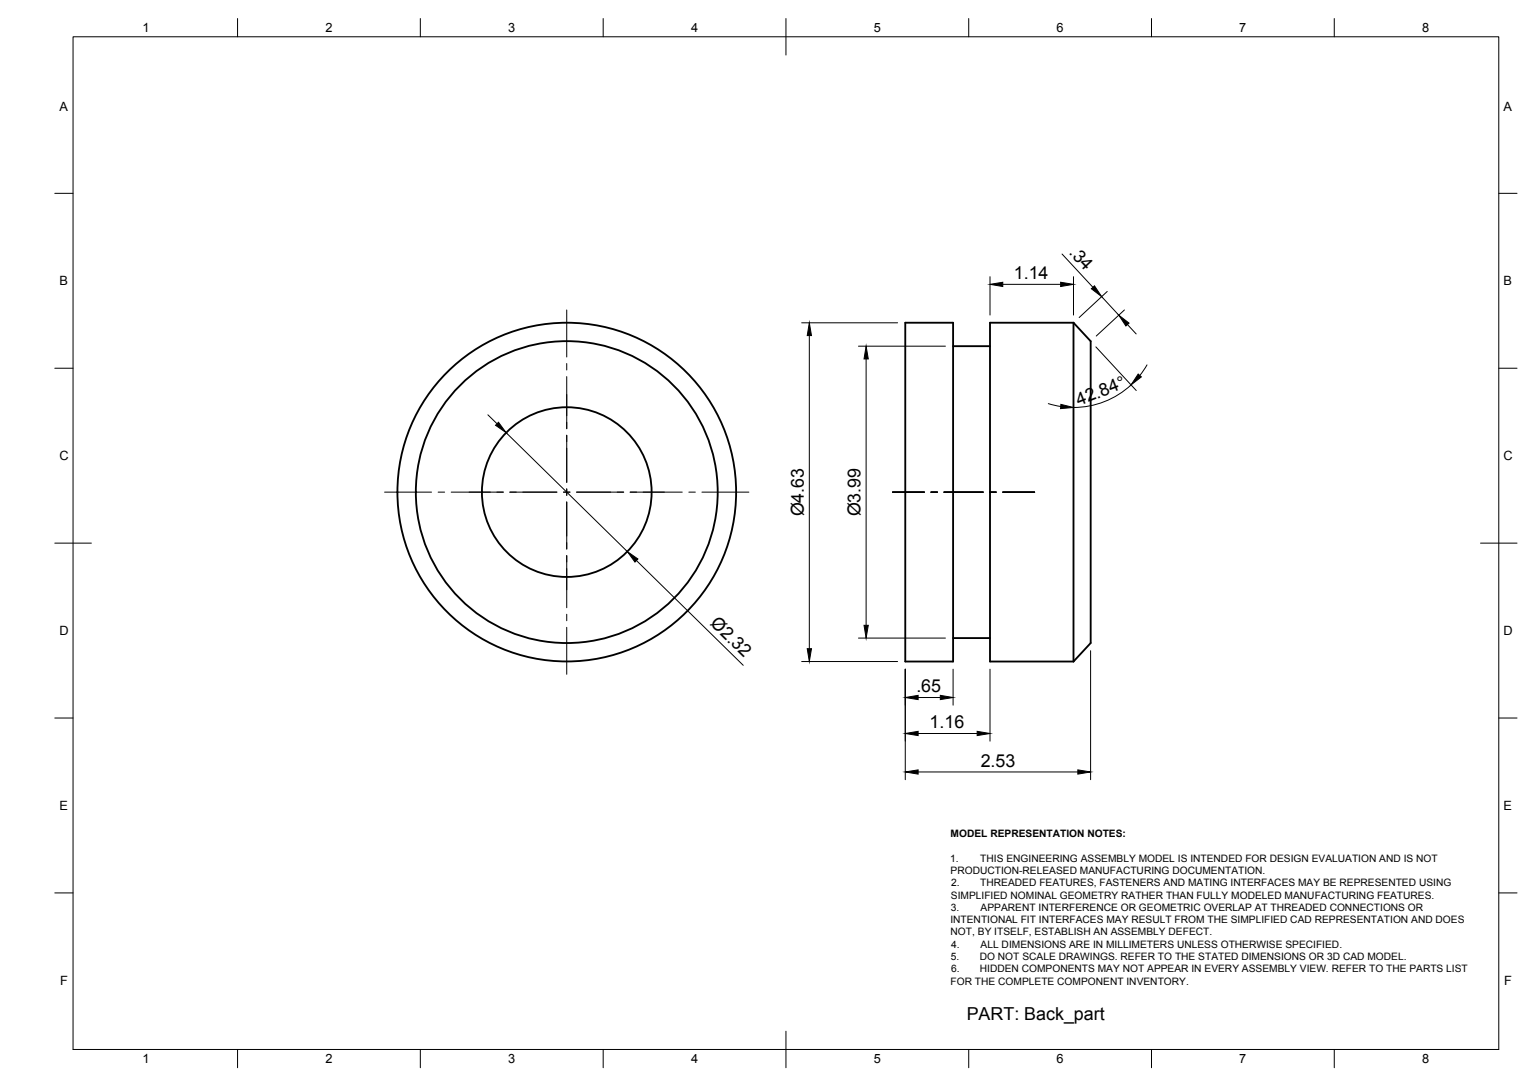
ISO-10303-21;
HEADER;
/* Generated by software containing ST-Developer
 * from STEP Tools, Inc. (www.steptools.com) 
 */

FILE_DESCRIPTION(
/* description */ (''),
/* implementation_level */ '2;1');

FILE_NAME(
/* name */ 'Back_part.step',
/* time_stamp */ '2026-10-05T00:51:14-07:00',
/* author */ (''),
/* organization */ (''),
/* preprocessor_version */ 'ST-DEVELOPER v20.2',
/* originating_system */ 'Autodesk Translation Framework v15.15.0.0',
/* authorisation */ '');

FILE_SCHEMA (('AUTOMOTIVE_DESIGN { 1 0 10303 214 3 1 1 }'));
ENDSEC;

DATA;
#10=MECHANICAL_DESIGN_GEOMETRIC_PRESENTATION_REPRESENTATION('',(#391),#4613);
#58=CONICAL_SURFACE('',#1792,2.1899902410121,0.823106104053138);
#59=CONICAL_SURFACE('',#1807,1.54725736664436,1.55720056407458);
#80=FACE_BOUND('',#574,.T.);
#81=FACE_BOUND('',#577,.T.);
#82=FACE_BOUND('',#580,.T.);
#83=FACE_BOUND('',#584,.T.);
#110=PLANE('',#1797);
#111=PLANE('',#1801);
#112=PLANE('',#1805);
#113=PLANE('',#1811);
#199=LINE('',#2684,#282);
#200=LINE('',#2689,#283);
#201=LINE('',#2696,#284);
#202=LINE('',#2703,#285);
#203=LINE('',#2710,#286);
#204=LINE('',#2714,#287);
#282=VECTOR('',#2142,2.1899902410121);
#283=VECTOR('',#2149,2.3164003912567);
#284=VECTOR('',#2158,1.99619194538056);
#285=VECTOR('',#2167,2.3164003912567);
#286=VECTOR('',#2176,1.54725736664436);
#287=VECTOR('',#2181,1.16083957311848);
#350=CYLINDRICAL_SURFACE('',#1795,2.3164003912567);
#351=CYLINDRICAL_SURFACE('',#1799,1.99619194538056);
#352=CYLINDRICAL_SURFACE('',#1803,2.3164003912567);
#353=CYLINDRICAL_SURFACE('',#1809,1.16083957311848);
#375=SHAPE_REPRESENTATION_RELATIONSHIP('SRR','None',#4649,#383);
#383=ADVANCED_BREP_SHAPE_REPRESENTATION('',(#399),#4609);
#391=STYLED_ITEM('',(#4695),#399);
#399=MANIFOLD_SOLID_BREP('Body1',#1598);
#452=FACE_OUTER_BOUND('',#571,.T.);
#453=FACE_OUTER_BOUND('',#572,.T.);
#454=FACE_OUTER_BOUND('',#573,.T.);
#455=FACE_OUTER_BOUND('',#575,.T.);
#456=FACE_OUTER_BOUND('',#576,.T.);
#457=FACE_OUTER_BOUND('',#578,.T.);
#458=FACE_OUTER_BOUND('',#579,.T.);
#459=FACE_OUTER_BOUND('',#581,.T.);
#460=FACE_OUTER_BOUND('',#582,.T.);
#461=FACE_OUTER_BOUND('',#583,.T.);
#571=EDGE_LOOP('',(#1245,#1246,#1247,#1248));
#572=EDGE_LOOP('',(#1249,#1250,#1251,#1252));
#573=EDGE_LOOP('',(#1253));
#574=EDGE_LOOP('',(#1254));
#575=EDGE_LOOP('',(#1255,#1256,#1257,#1258));
#576=EDGE_LOOP('',(#1259));
#577=EDGE_LOOP('',(#1260));
#578=EDGE_LOOP('',(#1261,#1262,#1263,#1264));
#579=EDGE_LOOP('',(#1265));
#580=EDGE_LOOP('',(#1266));
#581=EDGE_LOOP('',(#1267,#1268,#1269,#1270));
#582=EDGE_LOOP('',(#1271,#1272,#1273,#1274));
#583=EDGE_LOOP('',(#1275));
#584=EDGE_LOOP('',(#1276));
#685=CIRCLE('',#1793,2.3164003912567);
#686=CIRCLE('',#1794,2.06358009076751);
#687=CIRCLE('',#1796,2.3164003912567);
#688=CIRCLE('',#1798,1.99619194538056);
#689=CIRCLE('',#1800,1.99619194538056);
#690=CIRCLE('',#1802,2.3164003912567);
#691=CIRCLE('',#1804,2.3164003912567);
#692=CIRCLE('',#1806,1.93367516017024);
#693=CIRCLE('',#1808,1.16083957311848);
#694=CIRCLE('',#1810,1.16083957311848);
#786=VERTEX_POINT('',#2681);
#787=VERTEX_POINT('',#2683);
#788=VERTEX_POINT('',#2687);
#789=VERTEX_POINT('',#2691);
#790=VERTEX_POINT('',#2694);
#791=VERTEX_POINT('',#2698);
#792=VERTEX_POINT('',#2701);
#793=VERTEX_POINT('',#2705);
#794=VERTEX_POINT('',#2708);
#795=VERTEX_POINT('',#2712);
#950=EDGE_CURVE('',#786,#786,#685,.T.);
#951=EDGE_CURVE('',#786,#787,#199,.T.);
#952=EDGE_CURVE('',#787,#787,#686,.T.);
#953=EDGE_CURVE('',#788,#788,#687,.T.);
#954=EDGE_CURVE('',#788,#786,#200,.T.);
#955=EDGE_CURVE('',#789,#789,#688,.T.);
#956=EDGE_CURVE('',#790,#790,#689,.T.);
#957=EDGE_CURVE('',#790,#789,#201,.T.);
#958=EDGE_CURVE('',#791,#791,#690,.T.);
#959=EDGE_CURVE('',#792,#792,#691,.T.);
#960=EDGE_CURVE('',#792,#791,#202,.T.);
#961=EDGE_CURVE('',#793,#793,#692,.T.);
#962=EDGE_CURVE('',#794,#794,#693,.T.);
#963=EDGE_CURVE('',#794,#793,#203,.T.);
#964=EDGE_CURVE('',#795,#795,#694,.T.);
#965=EDGE_CURVE('',#795,#794,#204,.T.);
#1245=ORIENTED_EDGE('',*,*,#950,.F.);
#1246=ORIENTED_EDGE('',*,*,#951,.T.);
#1247=ORIENTED_EDGE('',*,*,#952,.T.);
#1248=ORIENTED_EDGE('',*,*,#951,.F.);
#1249=ORIENTED_EDGE('',*,*,#953,.F.);
#1250=ORIENTED_EDGE('',*,*,#954,.T.);
#1251=ORIENTED_EDGE('',*,*,#950,.T.);
#1252=ORIENTED_EDGE('',*,*,#954,.F.);
#1253=ORIENTED_EDGE('',*,*,#953,.T.);
#1254=ORIENTED_EDGE('',*,*,#955,.F.);
#1255=ORIENTED_EDGE('',*,*,#956,.F.);
#1256=ORIENTED_EDGE('',*,*,#957,.T.);
#1257=ORIENTED_EDGE('',*,*,#955,.T.);
#1258=ORIENTED_EDGE('',*,*,#957,.F.);
#1259=ORIENTED_EDGE('',*,*,#958,.F.);
#1260=ORIENTED_EDGE('',*,*,#956,.T.);
#1261=ORIENTED_EDGE('',*,*,#959,.F.);
#1262=ORIENTED_EDGE('',*,*,#960,.T.);
#1263=ORIENTED_EDGE('',*,*,#958,.T.);
#1264=ORIENTED_EDGE('',*,*,#960,.F.);
#1265=ORIENTED_EDGE('',*,*,#959,.T.);
#1266=ORIENTED_EDGE('',*,*,#961,.F.);
#1267=ORIENTED_EDGE('',*,*,#962,.F.);
#1268=ORIENTED_EDGE('',*,*,#963,.T.);
#1269=ORIENTED_EDGE('',*,*,#961,.T.);
#1270=ORIENTED_EDGE('',*,*,#963,.F.);
#1271=ORIENTED_EDGE('',*,*,#964,.F.);
#1272=ORIENTED_EDGE('',*,*,#965,.T.);
#1273=ORIENTED_EDGE('',*,*,#962,.T.);
#1274=ORIENTED_EDGE('',*,*,#965,.F.);
#1275=ORIENTED_EDGE('',*,*,#952,.F.);
#1276=ORIENTED_EDGE('',*,*,#964,.T.);
#1537=ADVANCED_FACE('',(#452),#58,.T.);
#1538=ADVANCED_FACE('',(#453),#350,.T.);
#1539=ADVANCED_FACE('',(#454,#80),#110,.T.);
#1540=ADVANCED_FACE('',(#455),#351,.T.);
#1541=ADVANCED_FACE('',(#456,#81),#111,.T.);
#1542=ADVANCED_FACE('',(#457),#352,.T.);
#1543=ADVANCED_FACE('',(#458,#82),#112,.T.);
#1544=ADVANCED_FACE('',(#459),#59,.F.);
#1545=ADVANCED_FACE('',(#460),#353,.F.);
#1546=ADVANCED_FACE('',(#461,#83),#113,.T.);
#1598=CLOSED_SHELL('',(#1537,#1538,#1539,#1540,#1541,#1542,#1543,#1544,
#1545,#1546));
#1791=AXIS2_PLACEMENT_3D('',#2679,#2136,#2137);
#1792=AXIS2_PLACEMENT_3D('',#2680,#2138,#2139);
#1793=AXIS2_PLACEMENT_3D('',#2682,#2140,#2141);
#1794=AXIS2_PLACEMENT_3D('',#2685,#2143,#2144);
#1795=AXIS2_PLACEMENT_3D('',#2686,#2145,#2146);
#1796=AXIS2_PLACEMENT_3D('',#2688,#2147,#2148);
#1797=AXIS2_PLACEMENT_3D('',#2690,#2150,#2151);
#1798=AXIS2_PLACEMENT_3D('',#2692,#2152,#2153);
#1799=AXIS2_PLACEMENT_3D('',#2693,#2154,#2155);
#1800=AXIS2_PLACEMENT_3D('',#2695,#2156,#2157);
#1801=AXIS2_PLACEMENT_3D('',#2697,#2159,#2160);
#1802=AXIS2_PLACEMENT_3D('',#2699,#2161,#2162);
#1803=AXIS2_PLACEMENT_3D('',#2700,#2163,#2164);
#1804=AXIS2_PLACEMENT_3D('',#2702,#2165,#2166);
#1805=AXIS2_PLACEMENT_3D('',#2704,#2168,#2169);
#1806=AXIS2_PLACEMENT_3D('',#2706,#2170,#2171);
#1807=AXIS2_PLACEMENT_3D('',#2707,#2172,#2173);
#1808=AXIS2_PLACEMENT_3D('',#2709,#2174,#2175);
#1809=AXIS2_PLACEMENT_3D('',#2711,#2177,#2178);
#1810=AXIS2_PLACEMENT_3D('',#2713,#2179,#2180);
#1811=AXIS2_PLACEMENT_3D('',#2715,#2182,#2183);
#2136=DIRECTION('axis',(0.,0.,1.));
#2137=DIRECTION('refdir',(1.,0.,0.));
#2138=DIRECTION('center_axis',(1.,0.,0.));
#2139=DIRECTION('ref_axis',(0.,0.,-1.));
#2140=DIRECTION('center_axis',(1.,0.,0.));
#2141=DIRECTION('ref_axis',(0.,0.,-1.));
#2142=DIRECTION('',(-0.67994690492187,8.97986164450499E-17,-0.733261349374948));
#2143=DIRECTION('center_axis',(1.,0.,0.));
#2144=DIRECTION('ref_axis',(0.,0.,-1.));
#2145=DIRECTION('center_axis',(1.,0.,0.));
#2146=DIRECTION('ref_axis',(0.,0.,-1.));
#2147=DIRECTION('center_axis',(1.,0.,0.));
#2148=DIRECTION('ref_axis',(0.,0.,-1.));
#2149=DIRECTION('',(-1.,0.,0.));
#2150=DIRECTION('center_axis',(1.,0.,0.));
#2151=DIRECTION('ref_axis',(0.,0.,-1.));
#2152=DIRECTION('center_axis',(1.,0.,0.));
#2153=DIRECTION('ref_axis',(0.,0.,-1.));
#2154=DIRECTION('center_axis',(1.,0.,0.));
#2155=DIRECTION('ref_axis',(0.,0.,-1.));
#2156=DIRECTION('center_axis',(1.,0.,0.));
#2157=DIRECTION('ref_axis',(0.,0.,-1.));
#2158=DIRECTION('',(-1.,0.,0.));
#2159=DIRECTION('center_axis',(-1.,0.,0.));
#2160=DIRECTION('ref_axis',(0.,0.,1.));
#2161=DIRECTION('center_axis',(1.,0.,0.));
#2162=DIRECTION('ref_axis',(0.,0.,-1.));
#2163=DIRECTION('center_axis',(1.,0.,0.));
#2164=DIRECTION('ref_axis',(0.,0.,-1.));
#2165=DIRECTION('center_axis',(1.,0.,0.));
#2166=DIRECTION('ref_axis',(0.,0.,-1.));
#2167=DIRECTION('',(-1.,0.,0.));
#2168=DIRECTION('center_axis',(1.,0.,0.));
#2169=DIRECTION('ref_axis',(0.,0.,-1.));
#2170=DIRECTION('center_axis',(1.,0.,0.));
#2171=DIRECTION('ref_axis',(0.,0.,-1.));
#2172=DIRECTION('center_axis',(1.,0.,0.));
#2173=DIRECTION('ref_axis',(0.,0.,-1.));
#2174=DIRECTION('center_axis',(1.,0.,0.));
#2175=DIRECTION('ref_axis',(0.,0.,-1.));
#2176=DIRECTION('',(0.0135953438732625,-1.22453361611656E-16,0.999907579041667));
#2177=DIRECTION('center_axis',(1.,0.,0.));
#2178=DIRECTION('ref_axis',(0.,0.,-1.));
#2179=DIRECTION('center_axis',(1.,0.,0.));
#2180=DIRECTION('ref_axis',(0.,0.,-1.));
#2181=DIRECTION('',(1.,0.,0.));
#2182=DIRECTION('center_axis',(-1.,0.,0.));
#2183=DIRECTION('ref_axis',(0.,0.,1.));
#2679=CARTESIAN_POINT('',(0.,0.,0.));
#2680=CARTESIAN_POINT('Origin',(-2.40309980332239,0.,0.));
#2681=CARTESIAN_POINT('',(-2.28588076473159,-2.83677232469619E-16,2.3164003912567));
#2682=CARTESIAN_POINT('Origin',(-2.28588076473159,0.,0.));
#2683=CARTESIAN_POINT('',(-2.52031884191318,-2.52715675294263E-16,2.06358009076751));
#2684=CARTESIAN_POINT('',(-2.40309980332239,-2.68196453881941E-16,2.1899902410121));
#2685=CARTESIAN_POINT('Origin',(-2.52031884191318,0.,0.));
#2686=CARTESIAN_POINT('Origin',(-1.71486702953379,0.,0.));
#2687=CARTESIAN_POINT('',(-1.14385329433599,-2.83677232469619E-16,2.3164003912567));
#2688=CARTESIAN_POINT('Origin',(-1.14385329433599,0.,0.));
#2689=CARTESIAN_POINT('',(-1.71486702953379,-2.83677232469619E-16,2.3164003912567));
#2690=CARTESIAN_POINT('Origin',(-1.14385329433599,0.,-1.99619194538056));
#2691=CARTESIAN_POINT('',(-1.14385329433599,-2.44463007639404E-16,1.99619194538056));
#2692=CARTESIAN_POINT('Origin',(-1.14385329433599,0.,0.));
#2693=CARTESIAN_POINT('Origin',(-0.89153499844287,0.,0.));
#2694=CARTESIAN_POINT('',(-0.639216702549746,-2.44463007639404E-16,1.99619194538056));
#2695=CARTESIAN_POINT('Origin',(-0.639216702549746,0.,0.));
#2696=CARTESIAN_POINT('',(-0.89153499844287,-2.44463007639403E-16,1.99619194538056));
#2697=CARTESIAN_POINT('Origin',(-0.639216702549746,0.,-2.3164003912567));
#2698=CARTESIAN_POINT('',(-0.639216702549746,-2.83677232469619E-16,2.3164003912567));
#2699=CARTESIAN_POINT('Origin',(-0.639216702549746,0.,0.));
#2700=CARTESIAN_POINT('Origin',(-0.312360226271176,0.,0.));
#2701=CARTESIAN_POINT('',(0.0144962500073953,-2.83677232469619E-16,2.3164003912567));
#2702=CARTESIAN_POINT('Origin',(0.0144962500073953,0.,0.));
#2703=CARTESIAN_POINT('',(-0.312360226271176,-2.83677232469619E-16,2.3164003912567));
#2704=CARTESIAN_POINT('Origin',(0.0144962500073953,0.,-1.93367516017024));
#2705=CARTESIAN_POINT('',(0.0144962500073953,-2.36806909549322E-16,1.93367516017024));
#2706=CARTESIAN_POINT('Origin',(0.0144962500073953,0.,0.));
#2707=CARTESIAN_POINT('Origin',(0.00924228164886909,0.,0.));
#2708=CARTESIAN_POINT('',(0.00398831329034288,-1.42161846754312E-16,1.16083957311848));
#2709=CARTESIAN_POINT('Origin',(0.00398831329034288,0.,0.));
#2710=CARTESIAN_POINT('',(0.00924228164886909,-1.89484378151818E-16,1.54725736664436));
#2711=CARTESIAN_POINT('Origin',(-1.25816526431142,0.,0.));
#2712=CARTESIAN_POINT('',(-2.52031884191318,-1.42161846754312E-16,1.16083957311848));
#2713=CARTESIAN_POINT('Origin',(-2.52031884191318,0.,0.));
#2714=CARTESIAN_POINT('',(-1.25816526431142,-1.42161846754313E-16,1.16083957311848));
#2715=CARTESIAN_POINT('Origin',(-2.52031884191318,0.,-2.06358009076751));
#4599=UNCERTAINTY_MEASURE_WITH_UNIT(LENGTH_MEASURE(0.01),#4614,
'DISTANCE_ACCURACY_VALUE',
'Maximum model space distance between geometric entities at asserted c
onnectivities');
#4603=UNCERTAINTY_MEASURE_WITH_UNIT(LENGTH_MEASURE(0.01),#4614,
'DISTANCE_ACCURACY_VALUE',
'Maximum model space distance between geometric entities at asserted c
onnectivities');
#4609=(
GEOMETRIC_REPRESENTATION_CONTEXT(3)
GLOBAL_UNCERTAINTY_ASSIGNED_CONTEXT((#4599))
GLOBAL_UNIT_ASSIGNED_CONTEXT((#4614,#4616,#4617))
REPRESENTATION_CONTEXT('','3D')
);
#4613=(
GEOMETRIC_REPRESENTATION_CONTEXT(3)
GLOBAL_UNCERTAINTY_ASSIGNED_CONTEXT((#4603))
GLOBAL_UNIT_ASSIGNED_CONTEXT((#4614,#4616,#4617))
REPRESENTATION_CONTEXT('','3D')
);
#4614=(
LENGTH_UNIT()
NAMED_UNIT(*)
SI_UNIT(.MILLI.,.METRE.)
);
#4616=(
NAMED_UNIT(*)
PLANE_ANGLE_UNIT()
SI_UNIT($,.RADIAN.)
);
#4617=(
NAMED_UNIT(*)
SI_UNIT($,.STERADIAN.)
SOLID_ANGLE_UNIT()
);
#4623=SHAPE_DEFINITION_REPRESENTATION(#4632,#4649);
#4632=PRODUCT_DEFINITION_SHAPE('',$,#4659);
#4649=SHAPE_REPRESENTATION('',(#1791),#4609);
#4653=PRODUCT_DEFINITION_CONTEXT('part definition',#4682,'design');
#4659=PRODUCT_DEFINITION('Back_part','Back_part',#4668,#4653);
#4668=PRODUCT_DEFINITION_FORMATION('',$,#4689);
#4682=APPLICATION_CONTEXT(
'Core Data for Automotive Mechanical Design Process');
#4683=PRODUCT_CONTEXT('part definition',#4682,'mechanical');
#4689=PRODUCT('Back_part','Back_part',$,(#4683));
#4695=PRESENTATION_STYLE_ASSIGNMENT((#4700));
#4700=SURFACE_STYLE_USAGE(.BOTH.,#4705);
#4705=SURFACE_SIDE_STYLE('',(#4710));
#4710=SURFACE_STYLE_FILL_AREA(#4715);
#4715=FILL_AREA_STYLE('Opaque(255,255,255)',(#4720));
#4720=FILL_AREA_STYLE_COLOUR('Opaque(255,255,255)',#4725);
#4725=COLOUR_RGB('Opaque(255,255,255)', 0.66274510, 0.83137255, 0.94901961);
ENDSEC;
END-ISO-10303-21;
